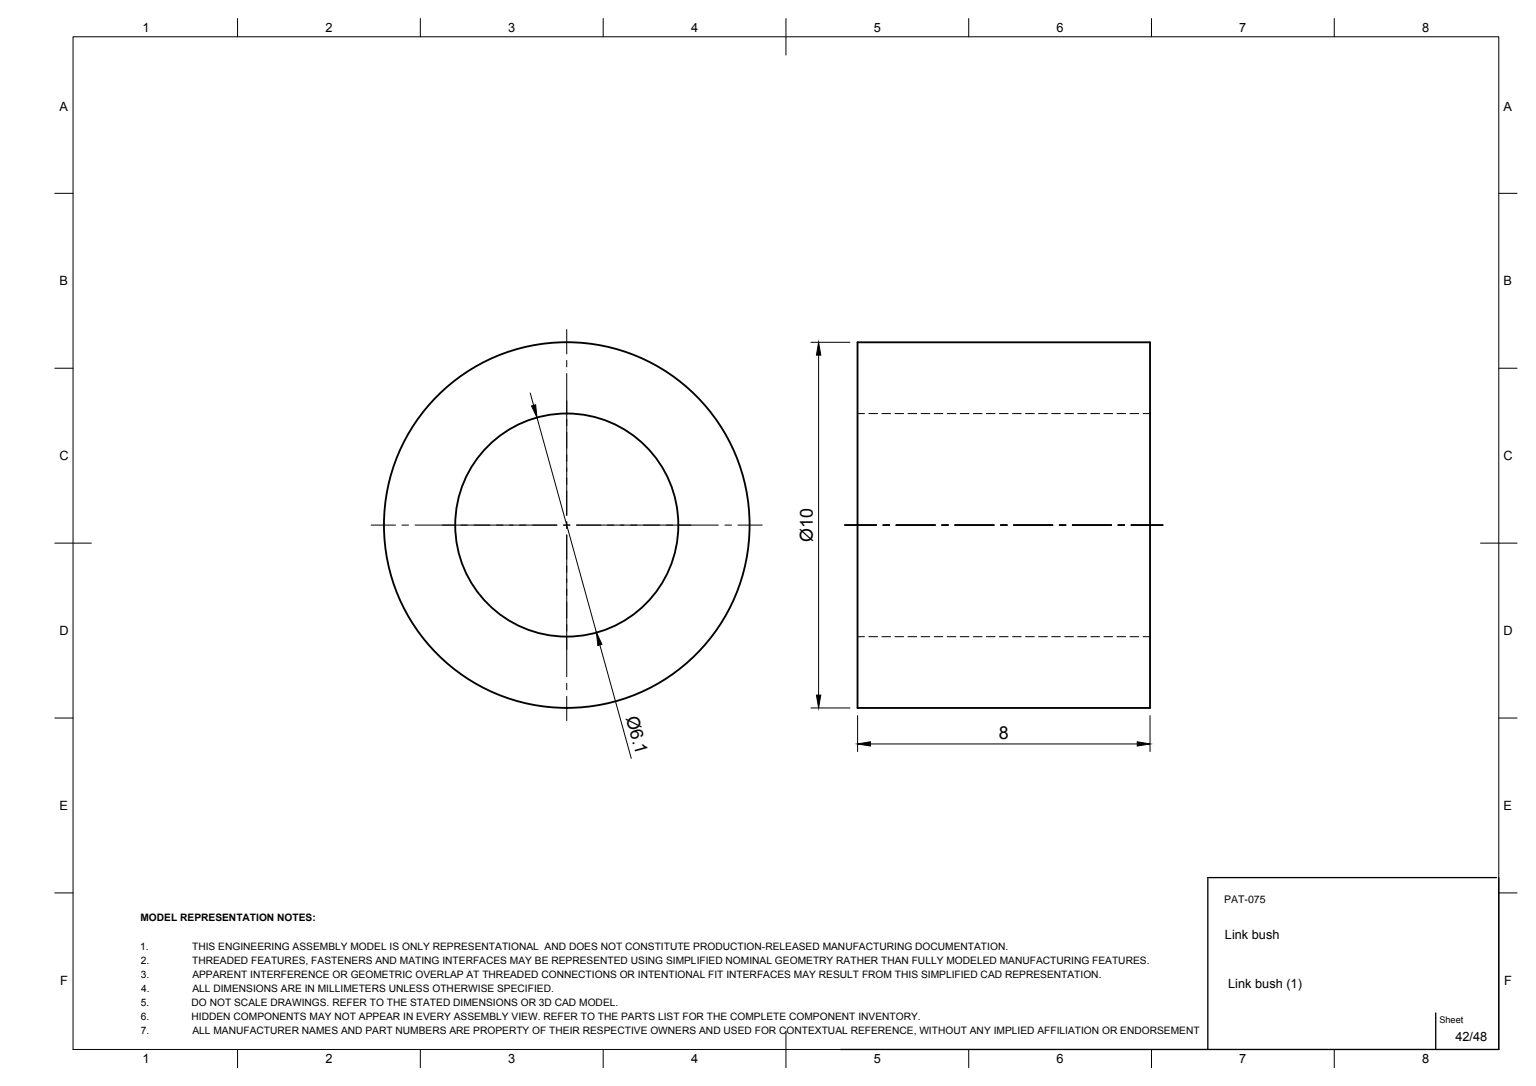
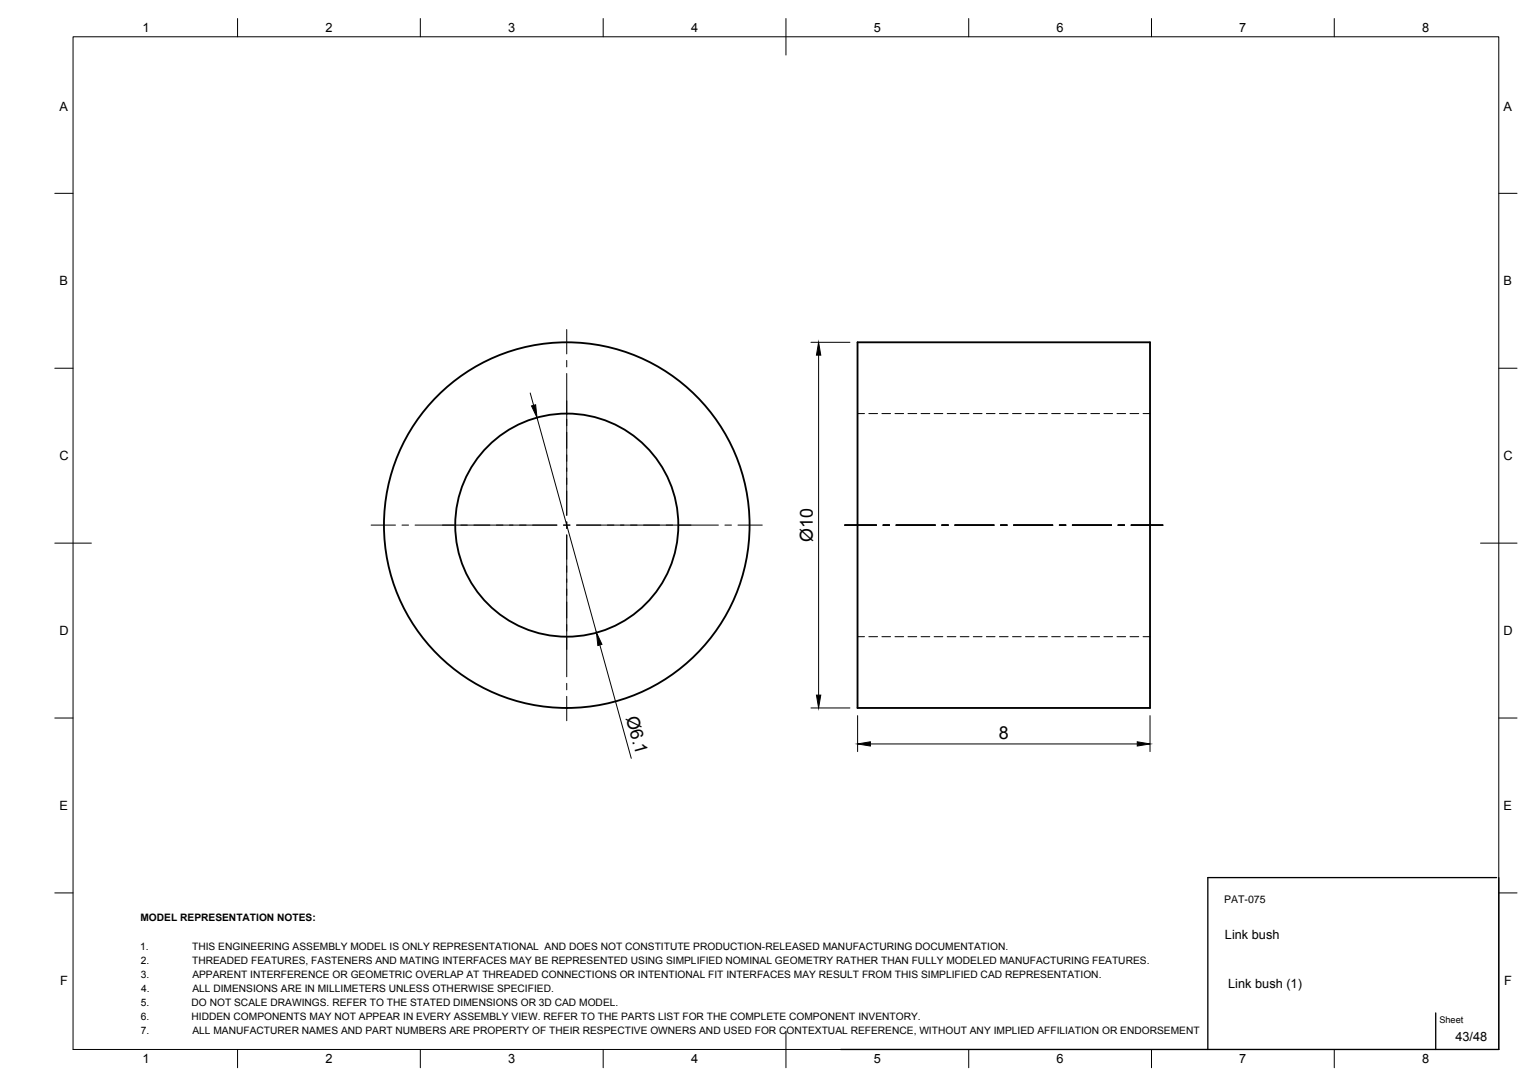
ISO-10303-21;
HEADER;
/* Generated by software containing ST-Developer
 * from STEP Tools, Inc. (www.steptools.com) 
 */

FILE_DESCRIPTION(
/* description */ ('Over-Centre Plunger Toggle Clamp on Slotted Fixture Frame'),
/* implementation_level */ '2;1');

FILE_NAME(
/* name */ 
'Link bush.step',
/* time_stamp */ '2026-10-28T03:23:24-07:00',
/* author */ (''),
/* organization */ (''),
/* preprocessor_version */ 'ST-DEVELOPER v20.2',
/* originating_system */ 'Autodesk Translation Framework v15.17.0.0',
/* authorisation */ '');

FILE_SCHEMA (('AUTOMOTIVE_DESIGN { 1 0 10303 214 3 1 1 }'));
ENDSEC;

DATA;
#10=MECHANICAL_DESIGN_GEOMETRIC_PRESENTATION_REPRESENTATION('',(#557),#15212);
#465=SHAPE_REPRESENTATION_RELATIONSHIP('SRR','None',#15443,#507);
#507=ADVANCED_BREP_SHAPE_REPRESENTATION('',(#604),#15205);
#557=STYLED_ITEM('',(#15733),#604);
#604=MANIFOLD_SOLID_BREP('Body1',#8293);
#772=FACE_BOUND('',#2171,.T.);
#773=FACE_BOUND('',#2173,.T.);
#1050=PLANE('',#9658);
#1051=PLANE('',#9659);
#1521=FACE_OUTER_BOUND('',#2168,.T.);
#1522=FACE_OUTER_BOUND('',#2169,.T.);
#1523=FACE_OUTER_BOUND('',#2170,.T.);
#1524=FACE_OUTER_BOUND('',#2172,.T.);
#2168=EDGE_LOOP('',(#7413,#7414,#7415,#7416));
#2169=EDGE_LOOP('',(#7417,#7418,#7419,#7420));
#2170=EDGE_LOOP('',(#7421));
#2171=EDGE_LOOP('',(#7422));
#2172=EDGE_LOOP('',(#7423));
#2173=EDGE_LOOP('',(#7424));
#2794=LINE('',#14861,#3424);
#2795=LINE('',#14867,#3425);
#3424=VECTOR('',#12099,0.305);
#3425=VECTOR('',#12106,0.5);
#3826=CIRCLE('',#9653,0.305);
#3827=CIRCLE('',#9654,0.305);
#3828=CIRCLE('',#9656,0.5);
#3829=CIRCLE('',#9657,0.5);
#4478=VERTEX_POINT('',#14858);
#4479=VERTEX_POINT('',#14860);
#4480=VERTEX_POINT('',#14864);
#4481=VERTEX_POINT('',#14866);
#5467=EDGE_CURVE('',#4478,#4478,#3826,.T.);
#5468=EDGE_CURVE('',#4478,#4479,#2794,.T.);
#5469=EDGE_CURVE('',#4479,#4479,#3827,.T.);
#5470=EDGE_CURVE('',#4480,#4480,#3828,.T.);
#5471=EDGE_CURVE('',#4480,#4481,#2795,.T.);
#5472=EDGE_CURVE('',#4481,#4481,#3829,.T.);
#7413=ORIENTED_EDGE('',*,*,#5467,.F.);
#7414=ORIENTED_EDGE('',*,*,#5468,.T.);
#7415=ORIENTED_EDGE('',*,*,#5469,.T.);
#7416=ORIENTED_EDGE('',*,*,#5468,.F.);
#7417=ORIENTED_EDGE('',*,*,#5470,.F.);
#7418=ORIENTED_EDGE('',*,*,#5471,.T.);
#7419=ORIENTED_EDGE('',*,*,#5472,.T.);
#7420=ORIENTED_EDGE('',*,*,#5471,.F.);
#7421=ORIENTED_EDGE('',*,*,#5470,.T.);
#7422=ORIENTED_EDGE('',*,*,#5467,.T.);
#7423=ORIENTED_EDGE('',*,*,#5472,.F.);
#7424=ORIENTED_EDGE('',*,*,#5469,.F.);
#7746=CYLINDRICAL_SURFACE('',#9652,0.305);
#7747=CYLINDRICAL_SURFACE('',#9655,0.5);
#8193=ADVANCED_FACE('',(#1521),#7746,.F.);
#8194=ADVANCED_FACE('',(#1522),#7747,.T.);
#8195=ADVANCED_FACE('',(#1523,#772),#1050,.T.);
#8196=ADVANCED_FACE('',(#1524,#773),#1051,.F.);
#8293=CLOSED_SHELL('',(#8193,#8194,#8195,#8196));
#9651=AXIS2_PLACEMENT_3D('',#14856,#12093,#12094);
#9652=AXIS2_PLACEMENT_3D('',#14857,#12095,#12096);
#9653=AXIS2_PLACEMENT_3D('',#14859,#12097,#12098);
#9654=AXIS2_PLACEMENT_3D('',#14862,#12100,#12101);
#9655=AXIS2_PLACEMENT_3D('',#14863,#12102,#12103);
#9656=AXIS2_PLACEMENT_3D('',#14865,#12104,#12105);
#9657=AXIS2_PLACEMENT_3D('',#14868,#12107,#12108);
#9658=AXIS2_PLACEMENT_3D('',#14869,#12109,#12110);
#9659=AXIS2_PLACEMENT_3D('',#14870,#12111,#12112);
#12093=DIRECTION('axis',(0.,0.,1.));
#12094=DIRECTION('refdir',(1.,0.,0.));
#12095=DIRECTION('center_axis',(0.,1.,0.));
#12096=DIRECTION('ref_axis',(1.,0.,0.));
#12097=DIRECTION('center_axis',(0.,-1.,0.));
#12098=DIRECTION('ref_axis',(1.,0.,0.));
#12099=DIRECTION('',(0.,-1.,0.));
#12100=DIRECTION('center_axis',(0.,-1.,0.));
#12101=DIRECTION('ref_axis',(1.,0.,0.));
#12102=DIRECTION('center_axis',(0.,1.,0.));
#12103=DIRECTION('ref_axis',(1.,0.,0.));
#12104=DIRECTION('center_axis',(0.,1.,0.));
#12105=DIRECTION('ref_axis',(1.,0.,0.));
#12106=DIRECTION('',(0.,-1.,0.));
#12107=DIRECTION('center_axis',(0.,1.,0.));
#12108=DIRECTION('ref_axis',(1.,0.,0.));
#12109=DIRECTION('center_axis',(0.,1.,0.));
#12110=DIRECTION('ref_axis',(1.,0.,0.));
#12111=DIRECTION('center_axis',(0.,1.,0.));
#12112=DIRECTION('ref_axis',(1.,0.,0.));
#14856=CARTESIAN_POINT('',(0.,0.,0.));
#14857=CARTESIAN_POINT('Origin',(-2.82632109303527,-5.5,8.79263101785268));
#14858=CARTESIAN_POINT('',(-3.13132109303527,-4.7,8.79263101785268));
#14859=CARTESIAN_POINT('Origin',(-2.82632109303527,-4.7,8.79263101785268));
#14860=CARTESIAN_POINT('',(-3.13132109303527,-5.5,8.79263101785268));
#14861=CARTESIAN_POINT('',(-3.13132109303527,-5.5,8.79263101785268));
#14862=CARTESIAN_POINT('Origin',(-2.82632109303527,-5.5,8.79263101785268));
#14863=CARTESIAN_POINT('Origin',(-2.82632109303527,-5.5,8.79263101785268));
#14864=CARTESIAN_POINT('',(-3.32632109303527,-4.7,8.79263101785268));
#14865=CARTESIAN_POINT('Origin',(-2.82632109303527,-4.7,8.79263101785268));
#14866=CARTESIAN_POINT('',(-3.32632109303527,-5.5,8.79263101785268));
#14867=CARTESIAN_POINT('',(-3.32632109303527,-5.5,8.79263101785268));
#14868=CARTESIAN_POINT('Origin',(-2.82632109303527,-5.5,8.79263101785268));
#14869=CARTESIAN_POINT('Origin',(-2.82632109303527,-4.7,8.79263101785268));
#14870=CARTESIAN_POINT('Origin',(-2.82632109303527,-5.5,8.79263101785268));
#15155=UNCERTAINTY_MEASURE_WITH_UNIT(LENGTH_MEASURE(0.001),#15213,
'DISTANCE_ACCURACY_VALUE',
'Maximum model space distance between geometric entities at asserted c
onnectivities');
#15162=UNCERTAINTY_MEASURE_WITH_UNIT(LENGTH_MEASURE(0.001),#15213,
'DISTANCE_ACCURACY_VALUE',
'Maximum model space distance between geometric entities at asserted c
onnectivities');
#15205=(
GEOMETRIC_REPRESENTATION_CONTEXT(3)
GLOBAL_UNCERTAINTY_ASSIGNED_CONTEXT((#15155))
GLOBAL_UNIT_ASSIGNED_CONTEXT((#15213,#15215,#15216))
REPRESENTATION_CONTEXT('','3D')
);
#15212=(
GEOMETRIC_REPRESENTATION_CONTEXT(3)
GLOBAL_UNCERTAINTY_ASSIGNED_CONTEXT((#15162))
GLOBAL_UNIT_ASSIGNED_CONTEXT((#15213,#15215,#15216))
REPRESENTATION_CONTEXT('','3D')
);
#15213=(
LENGTH_UNIT()
NAMED_UNIT(*)
SI_UNIT(.CENTI.,.METRE.)
);
#15215=(
NAMED_UNIT(*)
PLANE_ANGLE_UNIT()
SI_UNIT($,.RADIAN.)
);
#15216=(
NAMED_UNIT(*)
SI_UNIT($,.STERADIAN.)
SOLID_ANGLE_UNIT()
);
#15259=SHAPE_DEFINITION_REPRESENTATION(#15383,#15443);
#15383=PRODUCT_DEFINITION_SHAPE('',$,#15493);
#15443=SHAPE_REPRESENTATION('',(#9651),#15205);
#15450=PRODUCT_DEFINITION_CONTEXT('part definition',#15599,'design');
#15493=PRODUCT_DEFINITION('Link bush','Link bush',#15542,#15450);
#15542=PRODUCT_DEFINITION_FORMATION('',$,#15643);
#15599=APPLICATION_CONTEXT(
'Core Data for Automotive Mechanical Design Process');
#15600=PRODUCT_CONTEXT('part definition',#15599,'mechanical');
#15643=PRODUCT('Link bush','Link bush','Link bush',(#15600));
#15727=COLOUR_RGB('Off White',0.89,0.88,0.83);
#15728=FILL_AREA_STYLE_COLOUR('',#15727);
#15729=FILL_AREA_STYLE('',(#15728));
#15730=SURFACE_STYLE_FILL_AREA(#15729);
#15731=SURFACE_SIDE_STYLE('',(#15730));
#15732=SURFACE_STYLE_USAGE(.BOTH.,#15731);
#15733=PRESENTATION_STYLE_ASSIGNMENT((#15732));
ENDSEC;
END-ISO-10303-21;
